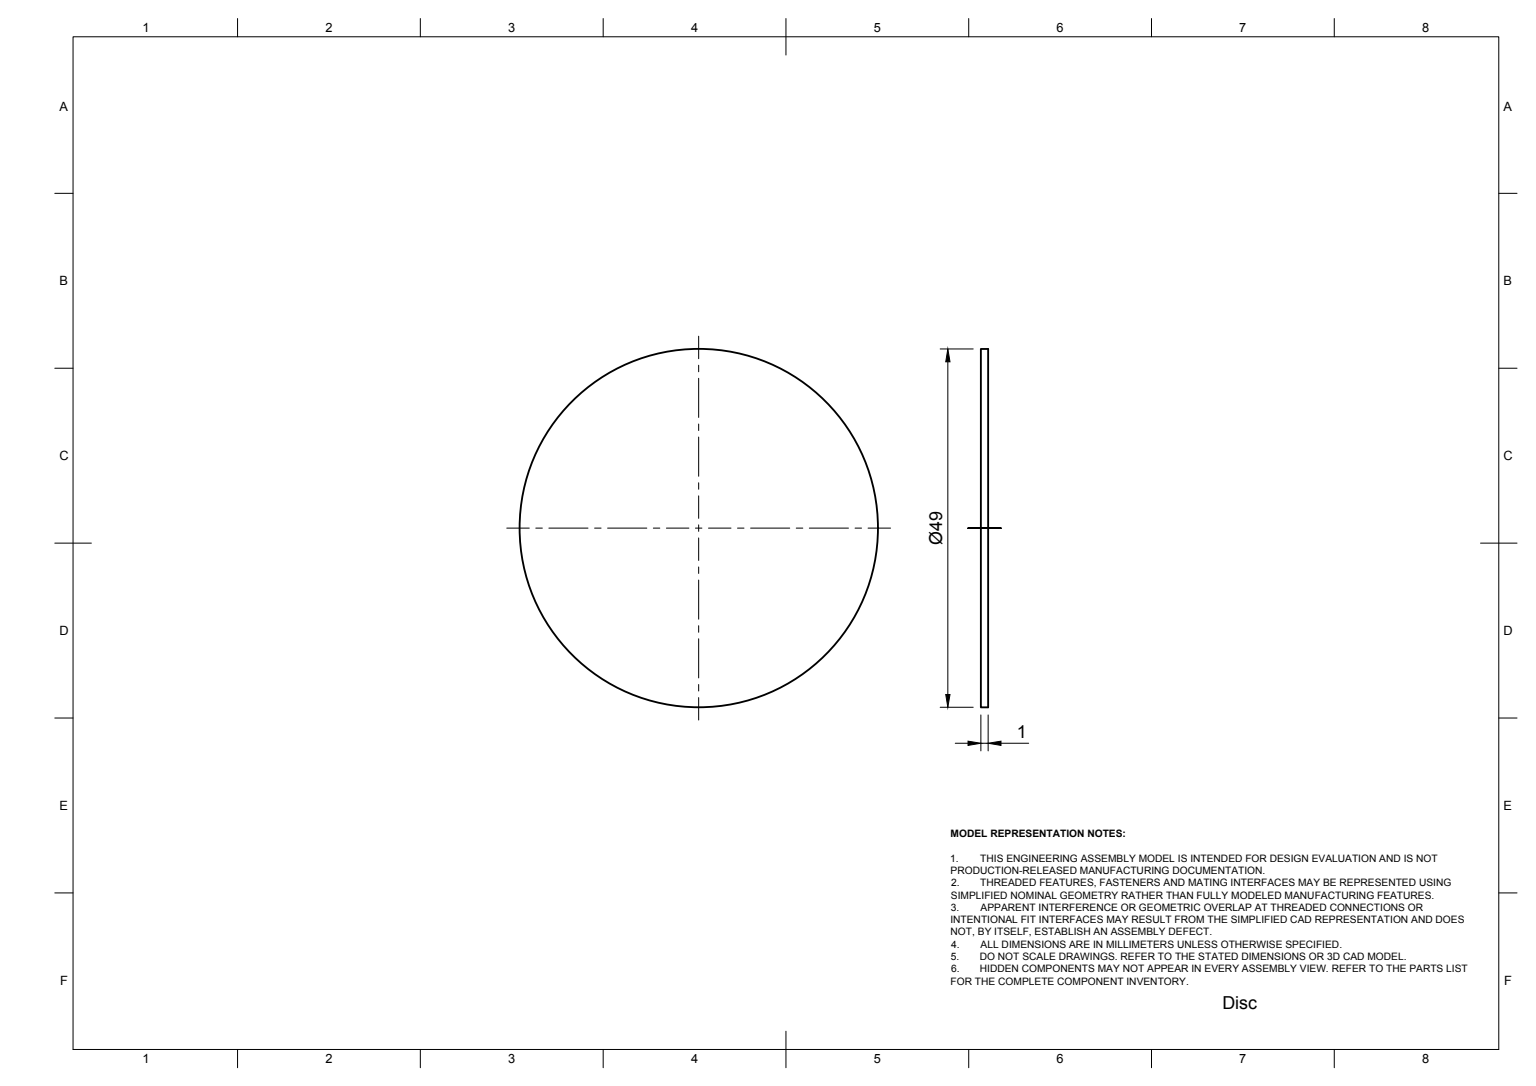
ISO-10303-21;
HEADER;
/* Generated by software containing ST-Developer
 * from STEP Tools, Inc. (www.steptools.com) 
 */

FILE_DESCRIPTION(
/* description */ (''),
/* implementation_level */ '2;1');

FILE_NAME(
/* name */ 'Disc.step',
/* time_stamp */ '2026-10-06T12:52:28-07:00',
/* author */ (''),
/* organization */ (''),
/* preprocessor_version */ 'ST-DEVELOPER v20.2',
/* originating_system */ 'Autodesk Translation Framework v15.15.0.0',
/* authorisation */ '');

FILE_SCHEMA (('AUTOMOTIVE_DESIGN { 1 0 10303 214 3 1 1 }'));
ENDSEC;

DATA;
#10=MECHANICAL_DESIGN_GEOMETRIC_PRESENTATION_REPRESENTATION('',(#74),#34403);
#58=SHAPE_REPRESENTATION_RELATIONSHIP('SRR','None',#34436,#66);
#66=ADVANCED_BREP_SHAPE_REPRESENTATION('',(#82),#34396);
#74=STYLED_ITEM('',(#34484),#82);
#82=MANIFOLD_SOLID_BREP('Body1',#4383);
#127=PLANE('',#4511);
#128=PLANE('',#4512);
#176=CIRCLE('',#4509,24.5);
#177=CIRCLE('',#4510,24.5);
#526=FACE_OUTER_BOUND('',#763,.T.);
#527=FACE_OUTER_BOUND('',#764,.T.);
#528=FACE_OUTER_BOUND('',#765,.T.);
#763=EDGE_LOOP('',(#2739,#2740,#2741,#2742));
#764=EDGE_LOOP('',(#2743));
#765=EDGE_LOOP('',(#2744));
#1018=LINE('',#6389,#1155);
#1155=VECTOR('',#5069,24.5);
#1560=VERTEX_POINT('',#6386);
#1561=VERTEX_POINT('',#6388);
#2034=EDGE_CURVE('',#1560,#1560,#176,.T.);
#2035=EDGE_CURVE('',#1560,#1561,#1018,.T.);
#2036=EDGE_CURVE('',#1561,#1561,#177,.T.);
#2739=ORIENTED_EDGE('',*,*,#2034,.F.);
#2740=ORIENTED_EDGE('',*,*,#2035,.T.);
#2741=ORIENTED_EDGE('',*,*,#2036,.F.);
#2742=ORIENTED_EDGE('',*,*,#2035,.F.);
#2743=ORIENTED_EDGE('',*,*,#2036,.T.);
#2744=ORIENTED_EDGE('',*,*,#2034,.T.);
#4041=CYLINDRICAL_SURFACE('',#4508,24.5);
#4161=ADVANCED_FACE('',(#526),#4041,.T.);
#4162=ADVANCED_FACE('',(#527),#127,.T.);
#4163=ADVANCED_FACE('',(#528),#128,.F.);
#4383=CLOSED_SHELL('',(#4161,#4162,#4163));
#4507=AXIS2_PLACEMENT_3D('',#6384,#5063,#5064);
#4508=AXIS2_PLACEMENT_3D('',#6385,#5065,#5066);
#4509=AXIS2_PLACEMENT_3D('',#6387,#5067,#5068);
#4510=AXIS2_PLACEMENT_3D('',#6390,#5070,#5071);
#4511=AXIS2_PLACEMENT_3D('',#6391,#5072,#5073);
#4512=AXIS2_PLACEMENT_3D('',#6392,#5074,#5075);
#5063=DIRECTION('axis',(0.,0.,1.));
#5064=DIRECTION('refdir',(1.,0.,0.));
#5065=DIRECTION('center_axis',(1.,2.22044604925031E-16,0.));
#5066=DIRECTION('ref_axis',(-2.22044604925031E-16,1.,0.));
#5067=DIRECTION('center_axis',(1.,2.22044604925031E-16,0.));
#5068=DIRECTION('ref_axis',(-2.22044604925031E-16,1.,0.));
#5069=DIRECTION('',(-1.,-2.22044604925031E-16,0.));
#5070=DIRECTION('center_axis',(-1.,-2.22044604925031E-16,0.));
#5071=DIRECTION('ref_axis',(-2.22044604925031E-16,1.,0.));
#5072=DIRECTION('center_axis',(-1.,-2.22044604925031E-16,0.));
#5073=DIRECTION('ref_axis',(-2.22044604925031E-16,1.,0.));
#5074=DIRECTION('center_axis',(-1.,-2.22044604925031E-16,0.));
#5075=DIRECTION('ref_axis',(-2.22044604925031E-16,1.,0.));
#6384=CARTESIAN_POINT('',(0.,0.,0.));
#6385=CARTESIAN_POINT('Origin',(-0.5,0.,0.));
#6386=CARTESIAN_POINT('',(0.500000000000005,-24.5,3.00038465791102E-15));
#6387=CARTESIAN_POINT('Origin',(0.5,2.22044604925031E-16,0.));
#6388=CARTESIAN_POINT('',(-0.499999999999995,-24.5,3.00038465791102E-15));
#6389=CARTESIAN_POINT('',(-0.499999999999995,-24.5,-3.00038465791102E-15));
#6390=CARTESIAN_POINT('Origin',(-0.5,0.,0.));
#6391=CARTESIAN_POINT('Origin',(-0.5,0.,0.));
#6392=CARTESIAN_POINT('Origin',(0.5,2.22044604925031E-16,0.));
#34386=UNCERTAINTY_MEASURE_WITH_UNIT(LENGTH_MEASURE(0.01),#34404,
'DISTANCE_ACCURACY_VALUE',
'Maximum model space distance between geometric entities at asserted c
onnectivities');
#34393=UNCERTAINTY_MEASURE_WITH_UNIT(LENGTH_MEASURE(0.01),#34404,
'DISTANCE_ACCURACY_VALUE',
'Maximum model space distance between geometric entities at asserted c
onnectivities');
#34396=(
GEOMETRIC_REPRESENTATION_CONTEXT(3)
GLOBAL_UNCERTAINTY_ASSIGNED_CONTEXT((#34386))
GLOBAL_UNIT_ASSIGNED_CONTEXT((#34404,#34406,#34407))
REPRESENTATION_CONTEXT('','3D')
);
#34403=(
GEOMETRIC_REPRESENTATION_CONTEXT(3)
GLOBAL_UNCERTAINTY_ASSIGNED_CONTEXT((#34393))
GLOBAL_UNIT_ASSIGNED_CONTEXT((#34404,#34406,#34407))
REPRESENTATION_CONTEXT('','3D')
);
#34404=(
LENGTH_UNIT()
NAMED_UNIT(*)
SI_UNIT(.MILLI.,.METRE.)
);
#34406=(
NAMED_UNIT(*)
PLANE_ANGLE_UNIT()
SI_UNIT($,.RADIAN.)
);
#34407=(
NAMED_UNIT(*)
SI_UNIT($,.STERADIAN.)
SOLID_ANGLE_UNIT()
);
#34410=SHAPE_DEFINITION_REPRESENTATION(#34419,#34436);
#34419=PRODUCT_DEFINITION_SHAPE('',$,#34446);
#34436=SHAPE_REPRESENTATION('',(#4507),#34396);
#34443=PRODUCT_DEFINITION_CONTEXT('part definition',#34472,'design');
#34446=PRODUCT_DEFINITION('Disc','Disc',#34455,#34443);
#34455=PRODUCT_DEFINITION_FORMATION('',$,#34476);
#34472=APPLICATION_CONTEXT(
'Core Data for Automotive Mechanical Design Process');
#34473=PRODUCT_CONTEXT('part definition',#34472,'mechanical');
#34476=PRODUCT('Disc','Disc',$,(#34473));
#34484=PRESENTATION_STYLE_ASSIGNMENT((#34486));
#34486=SURFACE_STYLE_USAGE(.BOTH.,#34488);
#34488=SURFACE_SIDE_STYLE('',(#34490));
#34490=SURFACE_STYLE_FILL_AREA(#34492);
#34492=FILL_AREA_STYLE('Opaque(160,160,160)',(#34494));
#34494=FILL_AREA_STYLE_COLOUR('Opaque(160,160,160)',#34496);
#34496=COLOUR_RGB('Opaque(160,160,160)', 0.09019608, 0.27058824, 0.51372549);
ENDSEC;
END-ISO-10303-21;
